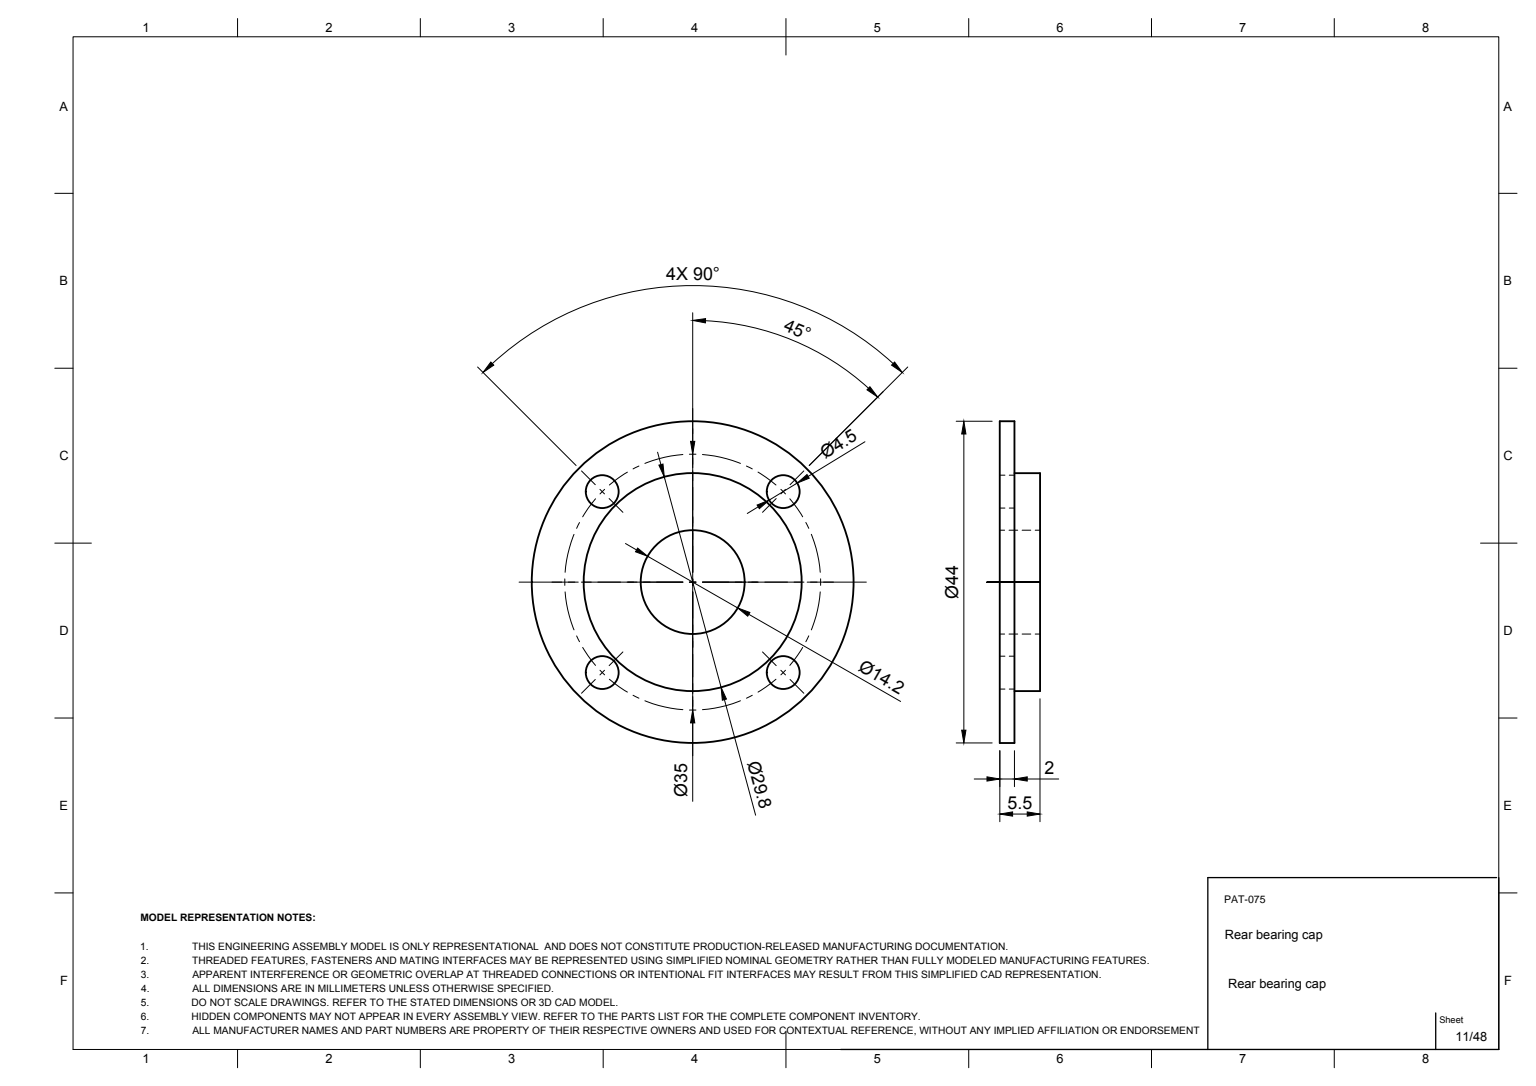
ISO-10303-21;
HEADER;
/* Generated by software containing ST-Developer
 * from STEP Tools, Inc. (www.steptools.com) 
 */

FILE_DESCRIPTION(
/* description */ ('Over-Centre Plunger Toggle Clamp on Slotted Fixture Frame'),
/* implementation_level */ '2;1');

FILE_NAME(
/* name */ 
'Rear bearing cap.step',
/* time_stamp */ '2026-10-28T03:23:24-07:00',
/* author */ (''),
/* organization */ (''),
/* preprocessor_version */ 'ST-DEVELOPER v20.2',
/* originating_system */ 'Autodesk Translation Framework v15.17.0.0',
/* authorisation */ '');

FILE_SCHEMA (('AUTOMOTIVE_DESIGN { 1 0 10303 214 3 1 1 }'));
ENDSEC;

DATA;
#10=MECHANICAL_DESIGN_GEOMETRIC_PRESENTATION_REPRESENTATION('',(#519),#15212);
#435=SHAPE_REPRESENTATION_RELATIONSHIP('SRR','None',#15409,#477);
#477=ADVANCED_BREP_SHAPE_REPRESENTATION('',(#570),#15171);
#519=STYLED_ITEM('',(#15719),#570);
#570=MANIFOLD_SOLID_BREP('Body1',#8251);
#682=FACE_BOUND('',#1738,.T.);
#683=FACE_BOUND('',#1742,.T.);
#684=FACE_BOUND('',#1743,.T.);
#685=FACE_BOUND('',#1744,.T.);
#686=FACE_BOUND('',#1745,.T.);
#687=FACE_BOUND('',#1746,.T.);
#688=FACE_BOUND('',#1748,.T.);
#689=FACE_BOUND('',#1749,.T.);
#690=FACE_BOUND('',#1750,.T.);
#691=FACE_BOUND('',#1751,.T.);
#692=FACE_BOUND('',#1752,.T.);
#830=PLANE('',#8957);
#831=PLANE('',#8964);
#832=PLANE('',#8965);
#1175=FACE_OUTER_BOUND('',#1732,.T.);
#1176=FACE_OUTER_BOUND('',#1733,.T.);
#1177=FACE_OUTER_BOUND('',#1734,.T.);
#1178=FACE_OUTER_BOUND('',#1735,.T.);
#1179=FACE_OUTER_BOUND('',#1736,.T.);
#1180=FACE_OUTER_BOUND('',#1737,.T.);
#1181=FACE_OUTER_BOUND('',#1739,.T.);
#1182=FACE_OUTER_BOUND('',#1740,.T.);
#1183=FACE_OUTER_BOUND('',#1741,.T.);
#1184=FACE_OUTER_BOUND('',#1747,.T.);
#1732=EDGE_LOOP('',(#5983,#5984,#5985,#5986));
#1733=EDGE_LOOP('',(#5987,#5988,#5989,#5990));
#1734=EDGE_LOOP('',(#5991,#5992,#5993,#5994));
#1735=EDGE_LOOP('',(#5995,#5996,#5997,#5998));
#1736=EDGE_LOOP('',(#5999,#6000,#6001,#6002));
#1737=EDGE_LOOP('',(#6003));
#1738=EDGE_LOOP('',(#6004));
#1739=EDGE_LOOP('',(#6005,#6006,#6007,#6008));
#1740=EDGE_LOOP('',(#6009,#6010,#6011,#6012));
#1741=EDGE_LOOP('',(#6013));
#1742=EDGE_LOOP('',(#6014));
#1743=EDGE_LOOP('',(#6015));
#1744=EDGE_LOOP('',(#6016));
#1745=EDGE_LOOP('',(#6017));
#1746=EDGE_LOOP('',(#6018));
#1747=EDGE_LOOP('',(#6019));
#1748=EDGE_LOOP('',(#6020));
#1749=EDGE_LOOP('',(#6021));
#1750=EDGE_LOOP('',(#6022));
#1751=EDGE_LOOP('',(#6023));
#1752=EDGE_LOOP('',(#6024));
#2356=LINE('',#12812,#2986);
#2357=LINE('',#12818,#2987);
#2358=LINE('',#12824,#2988);
#2359=LINE('',#12830,#2989);
#2360=LINE('',#12836,#2990);
#2361=LINE('',#12844,#2991);
#2362=LINE('',#12849,#2992);
#2986=VECTOR('',#10241,0.225);
#2987=VECTOR('',#10248,0.225);
#2988=VECTOR('',#10255,0.225);
#2989=VECTOR('',#10262,0.225);
#2990=VECTOR('',#10269,1.49);
#2991=VECTOR('',#10280,0.71);
#2992=VECTOR('',#10285,2.2);
#3573=CIRCLE('',#8943,0.225);
#3574=CIRCLE('',#8944,0.225);
#3575=CIRCLE('',#8946,0.225);
#3576=CIRCLE('',#8947,0.225);
#3577=CIRCLE('',#8949,0.225);
#3578=CIRCLE('',#8950,0.225);
#3579=CIRCLE('',#8952,0.225);
#3580=CIRCLE('',#8953,0.225);
#3581=CIRCLE('',#8955,1.49);
#3582=CIRCLE('',#8956,1.49);
#3583=CIRCLE('',#8958,0.71);
#3584=CIRCLE('',#8960,0.71);
#3585=CIRCLE('',#8962,2.2);
#3586=CIRCLE('',#8963,2.2);
#3997=VERTEX_POINT('',#12809);
#3998=VERTEX_POINT('',#12811);
#3999=VERTEX_POINT('',#12815);
#4000=VERTEX_POINT('',#12817);
#4001=VERTEX_POINT('',#12821);
#4002=VERTEX_POINT('',#12823);
#4003=VERTEX_POINT('',#12827);
#4004=VERTEX_POINT('',#12829);
#4005=VERTEX_POINT('',#12833);
#4006=VERTEX_POINT('',#12835);
#4007=VERTEX_POINT('',#12839);
#4008=VERTEX_POINT('',#12842);
#4009=VERTEX_POINT('',#12846);
#4010=VERTEX_POINT('',#12848);
#4752=EDGE_CURVE('',#3997,#3997,#3573,.T.);
#4753=EDGE_CURVE('',#3997,#3998,#2356,.T.);
#4754=EDGE_CURVE('',#3998,#3998,#3574,.T.);
#4755=EDGE_CURVE('',#3999,#3999,#3575,.T.);
#4756=EDGE_CURVE('',#3999,#4000,#2357,.T.);
#4757=EDGE_CURVE('',#4000,#4000,#3576,.T.);
#4758=EDGE_CURVE('',#4001,#4001,#3577,.T.);
#4759=EDGE_CURVE('',#4001,#4002,#2358,.T.);
#4760=EDGE_CURVE('',#4002,#4002,#3578,.T.);
#4761=EDGE_CURVE('',#4003,#4003,#3579,.T.);
#4762=EDGE_CURVE('',#4003,#4004,#2359,.T.);
#4763=EDGE_CURVE('',#4004,#4004,#3580,.T.);
#4764=EDGE_CURVE('',#4005,#4005,#3581,.T.);
#4765=EDGE_CURVE('',#4005,#4006,#2360,.T.);
#4766=EDGE_CURVE('',#4006,#4006,#3582,.T.);
#4767=EDGE_CURVE('',#4007,#4007,#3583,.T.);
#4768=EDGE_CURVE('',#4008,#4008,#3584,.T.);
#4769=EDGE_CURVE('',#4008,#4007,#2361,.T.);
#4770=EDGE_CURVE('',#4009,#4009,#3585,.T.);
#4771=EDGE_CURVE('',#4009,#4010,#2362,.T.);
#4772=EDGE_CURVE('',#4010,#4010,#3586,.T.);
#5983=ORIENTED_EDGE('',*,*,#4752,.F.);
#5984=ORIENTED_EDGE('',*,*,#4753,.T.);
#5985=ORIENTED_EDGE('',*,*,#4754,.F.);
#5986=ORIENTED_EDGE('',*,*,#4753,.F.);
#5987=ORIENTED_EDGE('',*,*,#4755,.F.);
#5988=ORIENTED_EDGE('',*,*,#4756,.T.);
#5989=ORIENTED_EDGE('',*,*,#4757,.F.);
#5990=ORIENTED_EDGE('',*,*,#4756,.F.);
#5991=ORIENTED_EDGE('',*,*,#4758,.F.);
#5992=ORIENTED_EDGE('',*,*,#4759,.T.);
#5993=ORIENTED_EDGE('',*,*,#4760,.F.);
#5994=ORIENTED_EDGE('',*,*,#4759,.F.);
#5995=ORIENTED_EDGE('',*,*,#4761,.F.);
#5996=ORIENTED_EDGE('',*,*,#4762,.T.);
#5997=ORIENTED_EDGE('',*,*,#4763,.F.);
#5998=ORIENTED_EDGE('',*,*,#4762,.F.);
#5999=ORIENTED_EDGE('',*,*,#4764,.F.);
#6000=ORIENTED_EDGE('',*,*,#4765,.T.);
#6001=ORIENTED_EDGE('',*,*,#4766,.T.);
#6002=ORIENTED_EDGE('',*,*,#4765,.F.);
#6003=ORIENTED_EDGE('',*,*,#4766,.F.);
#6004=ORIENTED_EDGE('',*,*,#4767,.F.);
#6005=ORIENTED_EDGE('',*,*,#4768,.F.);
#6006=ORIENTED_EDGE('',*,*,#4769,.T.);
#6007=ORIENTED_EDGE('',*,*,#4767,.T.);
#6008=ORIENTED_EDGE('',*,*,#4769,.F.);
#6009=ORIENTED_EDGE('',*,*,#4770,.F.);
#6010=ORIENTED_EDGE('',*,*,#4771,.T.);
#6011=ORIENTED_EDGE('',*,*,#4772,.T.);
#6012=ORIENTED_EDGE('',*,*,#4771,.F.);
#6013=ORIENTED_EDGE('',*,*,#4770,.T.);
#6014=ORIENTED_EDGE('',*,*,#4768,.T.);
#6015=ORIENTED_EDGE('',*,*,#4763,.T.);
#6016=ORIENTED_EDGE('',*,*,#4760,.T.);
#6017=ORIENTED_EDGE('',*,*,#4757,.T.);
#6018=ORIENTED_EDGE('',*,*,#4754,.T.);
#6019=ORIENTED_EDGE('',*,*,#4772,.F.);
#6020=ORIENTED_EDGE('',*,*,#4764,.T.);
#6021=ORIENTED_EDGE('',*,*,#4761,.T.);
#6022=ORIENTED_EDGE('',*,*,#4758,.T.);
#6023=ORIENTED_EDGE('',*,*,#4755,.T.);
#6024=ORIENTED_EDGE('',*,*,#4752,.T.);
#7658=CYLINDRICAL_SURFACE('',#8942,0.225);
#7659=CYLINDRICAL_SURFACE('',#8945,0.225);
#7660=CYLINDRICAL_SURFACE('',#8948,0.225);
#7661=CYLINDRICAL_SURFACE('',#8951,0.225);
#7662=CYLINDRICAL_SURFACE('',#8954,1.49);
#7663=CYLINDRICAL_SURFACE('',#8959,0.71);
#7664=CYLINDRICAL_SURFACE('',#8961,2.2);
#7847=ADVANCED_FACE('',(#1175),#7658,.F.);
#7848=ADVANCED_FACE('',(#1176),#7659,.F.);
#7849=ADVANCED_FACE('',(#1177),#7660,.F.);
#7850=ADVANCED_FACE('',(#1178),#7661,.F.);
#7851=ADVANCED_FACE('',(#1179),#7662,.T.);
#7852=ADVANCED_FACE('',(#1180,#682),#830,.F.);
#7853=ADVANCED_FACE('',(#1181),#7663,.F.);
#7854=ADVANCED_FACE('',(#1182),#7664,.T.);
#7855=ADVANCED_FACE('',(#1183,#683,#684,#685,#686,#687),#831,.T.);
#7856=ADVANCED_FACE('',(#1184,#688,#689,#690,#691,#692),#832,.F.);
#8251=CLOSED_SHELL('',(#7847,#7848,#7849,#7850,#7851,#7852,#7853,#7854,
#7855,#7856));
#8941=AXIS2_PLACEMENT_3D('',#12807,#10235,#10236);
#8942=AXIS2_PLACEMENT_3D('',#12808,#10237,#10238);
#8943=AXIS2_PLACEMENT_3D('',#12810,#10239,#10240);
#8944=AXIS2_PLACEMENT_3D('',#12813,#10242,#10243);
#8945=AXIS2_PLACEMENT_3D('',#12814,#10244,#10245);
#8946=AXIS2_PLACEMENT_3D('',#12816,#10246,#10247);
#8947=AXIS2_PLACEMENT_3D('',#12819,#10249,#10250);
#8948=AXIS2_PLACEMENT_3D('',#12820,#10251,#10252);
#8949=AXIS2_PLACEMENT_3D('',#12822,#10253,#10254);
#8950=AXIS2_PLACEMENT_3D('',#12825,#10256,#10257);
#8951=AXIS2_PLACEMENT_3D('',#12826,#10258,#10259);
#8952=AXIS2_PLACEMENT_3D('',#12828,#10260,#10261);
#8953=AXIS2_PLACEMENT_3D('',#12831,#10263,#10264);
#8954=AXIS2_PLACEMENT_3D('',#12832,#10265,#10266);
#8955=AXIS2_PLACEMENT_3D('',#12834,#10267,#10268);
#8956=AXIS2_PLACEMENT_3D('',#12837,#10270,#10271);
#8957=AXIS2_PLACEMENT_3D('',#12838,#10272,#10273);
#8958=AXIS2_PLACEMENT_3D('',#12840,#10274,#10275);
#8959=AXIS2_PLACEMENT_3D('',#12841,#10276,#10277);
#8960=AXIS2_PLACEMENT_3D('',#12843,#10278,#10279);
#8961=AXIS2_PLACEMENT_3D('',#12845,#10281,#10282);
#8962=AXIS2_PLACEMENT_3D('',#12847,#10283,#10284);
#8963=AXIS2_PLACEMENT_3D('',#12850,#10286,#10287);
#8964=AXIS2_PLACEMENT_3D('',#12851,#10288,#10289);
#8965=AXIS2_PLACEMENT_3D('',#12852,#10290,#10291);
#10235=DIRECTION('axis',(0.,0.,1.));
#10236=DIRECTION('refdir',(1.,0.,0.));
#10237=DIRECTION('center_axis',(0.,1.,0.));
#10238=DIRECTION('ref_axis',(1.,0.,0.));
#10239=DIRECTION('center_axis',(0.,1.,0.));
#10240=DIRECTION('ref_axis',(1.,0.,0.));
#10241=DIRECTION('',(0.,1.,0.));
#10242=DIRECTION('center_axis',(0.,-1.,0.));
#10243=DIRECTION('ref_axis',(1.,0.,0.));
#10244=DIRECTION('center_axis',(0.,1.,0.));
#10245=DIRECTION('ref_axis',(1.,0.,0.));
#10246=DIRECTION('center_axis',(0.,1.,0.));
#10247=DIRECTION('ref_axis',(1.,0.,0.));
#10248=DIRECTION('',(0.,1.,0.));
#10249=DIRECTION('center_axis',(0.,-1.,0.));
#10250=DIRECTION('ref_axis',(1.,0.,0.));
#10251=DIRECTION('center_axis',(0.,1.,0.));
#10252=DIRECTION('ref_axis',(1.,0.,0.));
#10253=DIRECTION('center_axis',(0.,1.,0.));
#10254=DIRECTION('ref_axis',(1.,0.,0.));
#10255=DIRECTION('',(0.,1.,0.));
#10256=DIRECTION('center_axis',(0.,-1.,0.));
#10257=DIRECTION('ref_axis',(1.,0.,0.));
#10258=DIRECTION('center_axis',(0.,1.,0.));
#10259=DIRECTION('ref_axis',(1.,0.,0.));
#10260=DIRECTION('center_axis',(0.,1.,0.));
#10261=DIRECTION('ref_axis',(1.,0.,0.));
#10262=DIRECTION('',(0.,1.,0.));
#10263=DIRECTION('center_axis',(0.,-1.,0.));
#10264=DIRECTION('ref_axis',(1.,0.,0.));
#10265=DIRECTION('center_axis',(0.,1.,0.));
#10266=DIRECTION('ref_axis',(1.,0.,0.));
#10267=DIRECTION('center_axis',(0.,1.,0.));
#10268=DIRECTION('ref_axis',(1.,0.,0.));
#10269=DIRECTION('',(0.,-1.,0.));
#10270=DIRECTION('center_axis',(0.,1.,0.));
#10271=DIRECTION('ref_axis',(1.,0.,0.));
#10272=DIRECTION('center_axis',(0.,1.,0.));
#10273=DIRECTION('ref_axis',(1.,0.,0.));
#10274=DIRECTION('center_axis',(0.,-1.,0.));
#10275=DIRECTION('ref_axis',(1.,0.,0.));
#10276=DIRECTION('center_axis',(0.,1.,0.));
#10277=DIRECTION('ref_axis',(1.,0.,0.));
#10278=DIRECTION('center_axis',(0.,-1.,0.));
#10279=DIRECTION('ref_axis',(1.,0.,0.));
#10280=DIRECTION('',(0.,-1.,0.));
#10281=DIRECTION('center_axis',(0.,1.,0.));
#10282=DIRECTION('ref_axis',(1.,0.,0.));
#10283=DIRECTION('center_axis',(0.,1.,0.));
#10284=DIRECTION('ref_axis',(1.,0.,0.));
#10285=DIRECTION('',(0.,-1.,0.));
#10286=DIRECTION('center_axis',(0.,1.,0.));
#10287=DIRECTION('ref_axis',(1.,0.,0.));
#10288=DIRECTION('center_axis',(0.,1.,0.));
#10289=DIRECTION('ref_axis',(1.,0.,0.));
#10290=DIRECTION('center_axis',(0.,1.,0.));
#10291=DIRECTION('ref_axis',(1.,0.,0.));
#12807=CARTESIAN_POINT('',(0.,0.,0.));
#12808=CARTESIAN_POINT('Origin',(-5.23743686707646,0.7,9.76256313292354));
#12809=CARTESIAN_POINT('',(-5.46243686707646,0.8,9.76256313292354));
#12810=CARTESIAN_POINT('Origin',(-5.23743686707646,0.8,9.76256313292354));
#12811=CARTESIAN_POINT('',(-5.46243686707646,1.,9.76256313292354));
#12812=CARTESIAN_POINT('',(-5.46243686707646,0.7,9.76256313292354));
#12813=CARTESIAN_POINT('Origin',(-5.23743686707646,1.,9.76256313292354));
#12814=CARTESIAN_POINT('Origin',(-5.23743686707646,0.7,12.2374368670765));
#12815=CARTESIAN_POINT('',(-5.46243686707646,0.8,12.2374368670765));
#12816=CARTESIAN_POINT('Origin',(-5.23743686707646,0.8,12.2374368670765));
#12817=CARTESIAN_POINT('',(-5.46243686707646,1.,12.2374368670765));
#12818=CARTESIAN_POINT('',(-5.46243686707646,0.7,12.2374368670765));
#12819=CARTESIAN_POINT('Origin',(-5.23743686707646,1.,12.2374368670765));
#12820=CARTESIAN_POINT('Origin',(-2.76256313292354,0.7,12.2374368670765));
#12821=CARTESIAN_POINT('',(-2.98756313292354,0.8,12.2374368670765));
#12822=CARTESIAN_POINT('Origin',(-2.76256313292354,0.8,12.2374368670765));
#12823=CARTESIAN_POINT('',(-2.98756313292354,1.,12.2374368670765));
#12824=CARTESIAN_POINT('',(-2.98756313292354,0.7,12.2374368670765));
#12825=CARTESIAN_POINT('Origin',(-2.76256313292354,1.,12.2374368670765));
#12826=CARTESIAN_POINT('Origin',(-2.76256313292354,0.7,9.76256313292354));
#12827=CARTESIAN_POINT('',(-2.98756313292354,0.8,9.76256313292354));
#12828=CARTESIAN_POINT('Origin',(-2.76256313292354,0.8,9.76256313292354));
#12829=CARTESIAN_POINT('',(-2.98756313292354,1.,9.76256313292354));
#12830=CARTESIAN_POINT('',(-2.98756313292354,0.7,9.76256313292354));
#12831=CARTESIAN_POINT('Origin',(-2.76256313292354,1.,9.76256313292354));
#12832=CARTESIAN_POINT('Origin',(-4.,0.45,11.));
#12833=CARTESIAN_POINT('',(-5.49,0.8,11.));
#12834=CARTESIAN_POINT('Origin',(-4.,0.8,11.));
#12835=CARTESIAN_POINT('',(-5.49,0.45,11.));
#12836=CARTESIAN_POINT('',(-5.49,0.45,11.));
#12837=CARTESIAN_POINT('Origin',(-4.,0.45,11.));
#12838=CARTESIAN_POINT('Origin',(-4.,0.45,11.));
#12839=CARTESIAN_POINT('',(-4.71,0.45,11.));
#12840=CARTESIAN_POINT('Origin',(-4.,0.45,11.));
#12841=CARTESIAN_POINT('Origin',(-4.,0.8,11.));
#12842=CARTESIAN_POINT('',(-4.71,1.,11.));
#12843=CARTESIAN_POINT('Origin',(-4.,1.,11.));
#12844=CARTESIAN_POINT('',(-4.71,0.8,11.));
#12845=CARTESIAN_POINT('Origin',(-4.,0.8,11.));
#12846=CARTESIAN_POINT('',(-6.2,1.,11.));
#12847=CARTESIAN_POINT('Origin',(-4.,1.,11.));
#12848=CARTESIAN_POINT('',(-6.2,0.8,11.));
#12849=CARTESIAN_POINT('',(-6.2,0.8,11.));
#12850=CARTESIAN_POINT('Origin',(-4.,0.8,11.));
#12851=CARTESIAN_POINT('Origin',(-4.,1.,11.));
#12852=CARTESIAN_POINT('Origin',(-4.,0.8,11.));
#15121=UNCERTAINTY_MEASURE_WITH_UNIT(LENGTH_MEASURE(0.001),#15213,
'DISTANCE_ACCURACY_VALUE',
'Maximum model space distance between geometric entities at asserted c
onnectivities');
#15162=UNCERTAINTY_MEASURE_WITH_UNIT(LENGTH_MEASURE(0.001),#15213,
'DISTANCE_ACCURACY_VALUE',
'Maximum model space distance between geometric entities at asserted c
onnectivities');
#15171=(
GEOMETRIC_REPRESENTATION_CONTEXT(3)
GLOBAL_UNCERTAINTY_ASSIGNED_CONTEXT((#15121))
GLOBAL_UNIT_ASSIGNED_CONTEXT((#15213,#15215,#15216))
REPRESENTATION_CONTEXT('','3D')
);
#15212=(
GEOMETRIC_REPRESENTATION_CONTEXT(3)
GLOBAL_UNCERTAINTY_ASSIGNED_CONTEXT((#15162))
GLOBAL_UNIT_ASSIGNED_CONTEXT((#15213,#15215,#15216))
REPRESENTATION_CONTEXT('','3D')
);
#15213=(
LENGTH_UNIT()
NAMED_UNIT(*)
SI_UNIT(.CENTI.,.METRE.)
);
#15215=(
NAMED_UNIT(*)
PLANE_ANGLE_UNIT()
SI_UNIT($,.RADIAN.)
);
#15216=(
NAMED_UNIT(*)
SI_UNIT($,.STERADIAN.)
SOLID_ANGLE_UNIT()
);
#15225=SHAPE_DEFINITION_REPRESENTATION(#15274,#15409);
#15274=PRODUCT_DEFINITION_SHAPE('',$,#15459);
#15409=SHAPE_REPRESENTATION('',(#8941),#15171);
#15450=PRODUCT_DEFINITION_CONTEXT('part definition',#15599,'design');
#15459=PRODUCT_DEFINITION('Rear bearing cap','Rear bearing cap',#15508,
#15450);
#15508=PRODUCT_DEFINITION_FORMATION('',$,#15609);
#15599=APPLICATION_CONTEXT(
'Core Data for Automotive Mechanical Design Process');
#15600=PRODUCT_CONTEXT('part definition',#15599,'mechanical');
#15609=PRODUCT('Rear bearing cap','Rear bearing cap','Rear bearing cap',
(#15600));
#15713=COLOUR_RGB('Grey',0.48,0.52,0.57);
#15714=FILL_AREA_STYLE_COLOUR('',#15713);
#15715=FILL_AREA_STYLE('',(#15714));
#15716=SURFACE_STYLE_FILL_AREA(#15715);
#15717=SURFACE_SIDE_STYLE('',(#15716));
#15718=SURFACE_STYLE_USAGE(.BOTH.,#15717);
#15719=PRESENTATION_STYLE_ASSIGNMENT((#15718));
ENDSEC;
END-ISO-10303-21;
